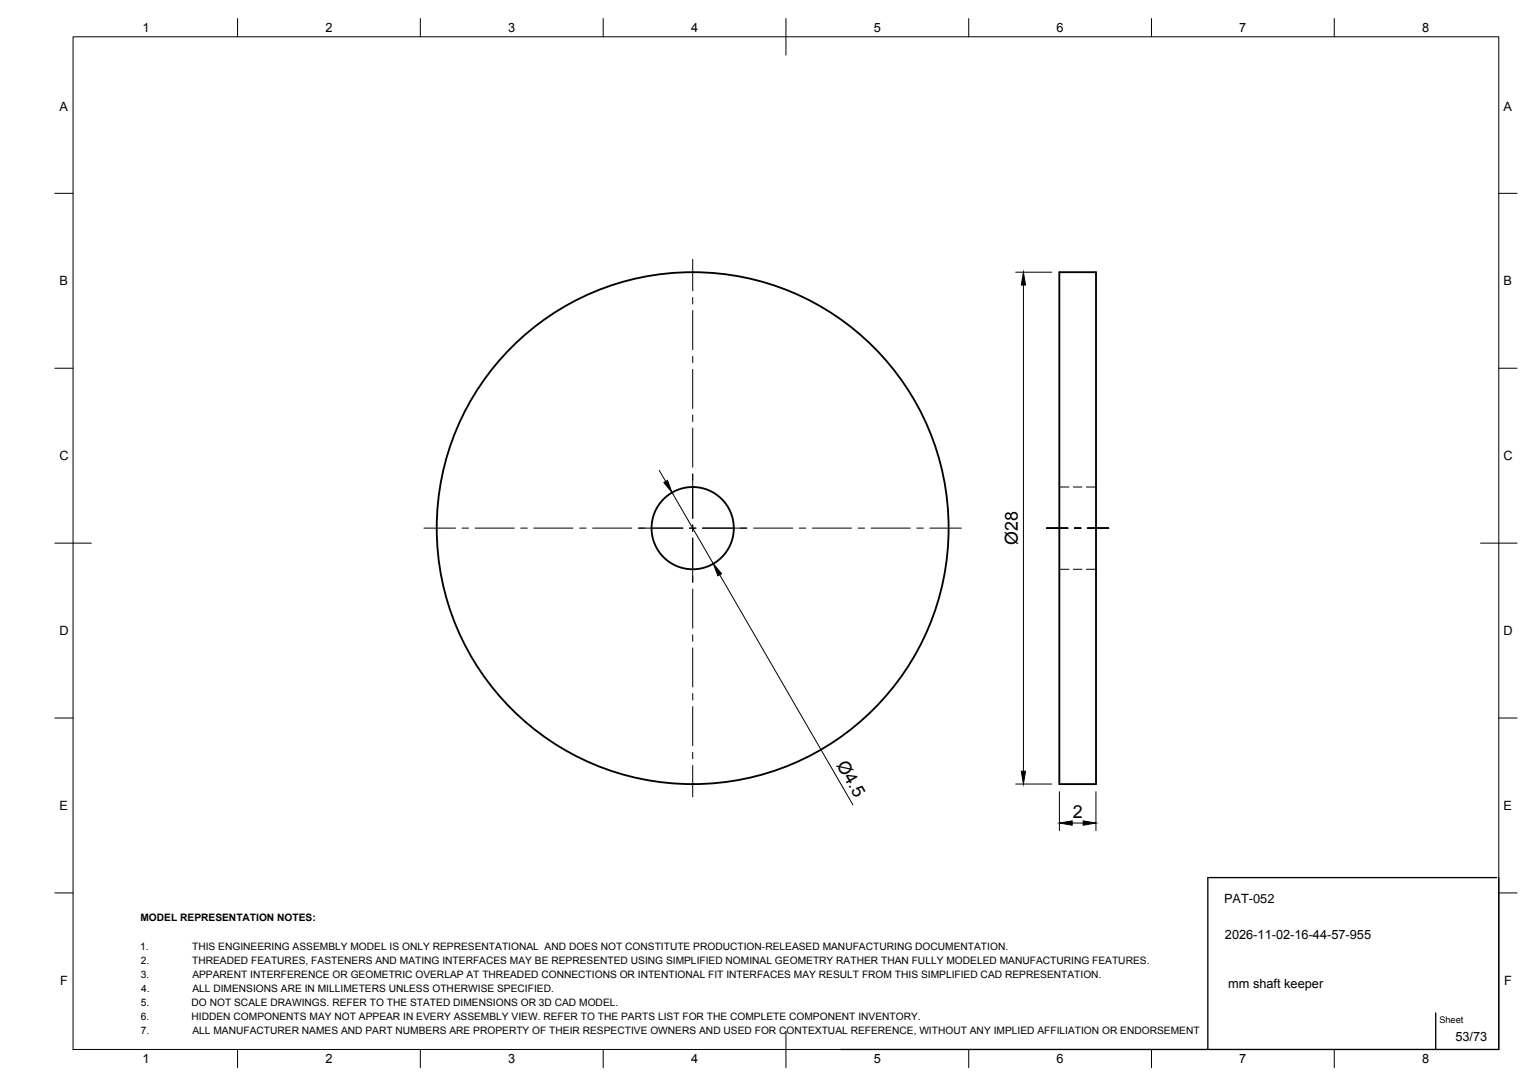
ISO-10303-21;
HEADER;
/* Generated by software containing ST-Developer
 * from STEP Tools, Inc. (www.steptools.com) 
 */

FILE_DESCRIPTION(
/* description */ ('Hand-crank gear train demonstrator'),
/* implementation_level */ '2;1');

FILE_NAME(
/* name */ 'mm shaft keeper.step',
/* time_stamp */ '2026-10-28T03:22:13-07:00',
/* author */ (''),
/* organization */ (''),
/* preprocessor_version */ 'ST-DEVELOPER v20.2',
/* originating_system */ 'Autodesk Translation Framework v15.17.0.0',
/* authorisation */ '');

FILE_SCHEMA (('AUTOMOTIVE_DESIGN { 1 0 10303 214 3 1 1 }'));
ENDSEC;

DATA;
#10=MECHANICAL_DESIGN_GEOMETRIC_PRESENTATION_REPRESENTATION('',(#1247),#62758);
#1104=SHAPE_REPRESENTATION_RELATIONSHIP('SRR','None',#63080,#1168);
#1168=ADVANCED_BREP_SHAPE_REPRESENTATION('',(#1322),#62734);
#1247=STYLED_ITEM('',(#63462),#1322);
#1322=MANIFOLD_SOLID_BREP('Body1',#16431);
#1584=FACE_BOUND('',#3842,.T.);
#1585=FACE_BOUND('',#3844,.T.);
#1955=PLANE('',#18201);
#1956=PLANE('',#18202);
#2661=FACE_OUTER_BOUND('',#3839,.T.);
#2662=FACE_OUTER_BOUND('',#3840,.T.);
#2663=FACE_OUTER_BOUND('',#3841,.T.);
#2664=FACE_OUTER_BOUND('',#3843,.T.);
#3839=EDGE_LOOP('',(#13127,#13128,#13129,#13130));
#3840=EDGE_LOOP('',(#13131,#13132,#13133,#13134));
#3841=EDGE_LOOP('',(#13135));
#3842=EDGE_LOOP('',(#13136));
#3843=EDGE_LOOP('',(#13137));
#3844=EDGE_LOOP('',(#13138));
#4953=LINE('',#26579,#6085);
#4954=LINE('',#26585,#6086);
#6085=VECTOR('',#21576,0.225);
#6086=VECTOR('',#21583,1.4);
#6989=CIRCLE('',#18196,0.225);
#6990=CIRCLE('',#18197,0.225);
#6991=CIRCLE('',#18199,1.4);
#6992=CIRCLE('',#18200,1.4);
#7990=VERTEX_POINT('',#26576);
#7991=VERTEX_POINT('',#26578);
#7992=VERTEX_POINT('',#26582);
#7993=VERTEX_POINT('',#26584);
#9815=EDGE_CURVE('',#7990,#7990,#6989,.T.);
#9816=EDGE_CURVE('',#7990,#7991,#4953,.T.);
#9817=EDGE_CURVE('',#7991,#7991,#6990,.T.);
#9818=EDGE_CURVE('',#7992,#7992,#6991,.T.);
#9819=EDGE_CURVE('',#7992,#7993,#4954,.T.);
#9820=EDGE_CURVE('',#7993,#7993,#6992,.T.);
#13127=ORIENTED_EDGE('',*,*,#9815,.F.);
#13128=ORIENTED_EDGE('',*,*,#9816,.T.);
#13129=ORIENTED_EDGE('',*,*,#9817,.T.);
#13130=ORIENTED_EDGE('',*,*,#9816,.F.);
#13131=ORIENTED_EDGE('',*,*,#9818,.F.);
#13132=ORIENTED_EDGE('',*,*,#9819,.T.);
#13133=ORIENTED_EDGE('',*,*,#9820,.T.);
#13134=ORIENTED_EDGE('',*,*,#9819,.F.);
#13135=ORIENTED_EDGE('',*,*,#9818,.T.);
#13136=ORIENTED_EDGE('',*,*,#9815,.T.);
#13137=ORIENTED_EDGE('',*,*,#9820,.F.);
#13138=ORIENTED_EDGE('',*,*,#9817,.F.);
#15329=CYLINDRICAL_SURFACE('',#18195,0.225);
#15330=CYLINDRICAL_SURFACE('',#18198,1.4);
#15971=ADVANCED_FACE('',(#2661),#15329,.F.);
#15972=ADVANCED_FACE('',(#2662),#15330,.T.);
#15973=ADVANCED_FACE('',(#2663,#1584),#1955,.T.);
#15974=ADVANCED_FACE('',(#2664,#1585),#1956,.F.);
#16431=CLOSED_SHELL('',(#15971,#15972,#15973,#15974));
#18194=AXIS2_PLACEMENT_3D('',#26574,#21570,#21571);
#18195=AXIS2_PLACEMENT_3D('',#26575,#21572,#21573);
#18196=AXIS2_PLACEMENT_3D('',#26577,#21574,#21575);
#18197=AXIS2_PLACEMENT_3D('',#26580,#21577,#21578);
#18198=AXIS2_PLACEMENT_3D('',#26581,#21579,#21580);
#18199=AXIS2_PLACEMENT_3D('',#26583,#21581,#21582);
#18200=AXIS2_PLACEMENT_3D('',#26586,#21584,#21585);
#18201=AXIS2_PLACEMENT_3D('',#26587,#21586,#21587);
#18202=AXIS2_PLACEMENT_3D('',#26588,#21588,#21589);
#21570=DIRECTION('axis',(0.,0.,1.));
#21571=DIRECTION('refdir',(1.,0.,0.));
#21572=DIRECTION('center_axis',(0.,1.,0.));
#21573=DIRECTION('ref_axis',(1.,0.,0.));
#21574=DIRECTION('center_axis',(0.,-1.,0.));
#21575=DIRECTION('ref_axis',(1.,0.,0.));
#21576=DIRECTION('',(0.,-1.,0.));
#21577=DIRECTION('center_axis',(0.,-1.,0.));
#21578=DIRECTION('ref_axis',(1.,0.,0.));
#21579=DIRECTION('center_axis',(0.,1.,0.));
#21580=DIRECTION('ref_axis',(1.,0.,0.));
#21581=DIRECTION('center_axis',(0.,1.,0.));
#21582=DIRECTION('ref_axis',(1.,0.,0.));
#21583=DIRECTION('',(0.,-1.,0.));
#21584=DIRECTION('center_axis',(0.,1.,0.));
#21585=DIRECTION('ref_axis',(1.,0.,0.));
#21586=DIRECTION('center_axis',(0.,1.,0.));
#21587=DIRECTION('ref_axis',(1.,0.,0.));
#21588=DIRECTION('center_axis',(0.,1.,0.));
#21589=DIRECTION('ref_axis',(1.,0.,0.));
#26574=CARTESIAN_POINT('',(0.,0.,0.));
#26575=CARTESIAN_POINT('Origin',(6.,3.2,9.));
#26576=CARTESIAN_POINT('',(5.775,3.4,9.));
#26577=CARTESIAN_POINT('Origin',(6.,3.4,9.));
#26578=CARTESIAN_POINT('',(5.775,3.2,9.));
#26579=CARTESIAN_POINT('',(5.775,3.2,9.));
#26580=CARTESIAN_POINT('Origin',(6.,3.2,9.));
#26581=CARTESIAN_POINT('Origin',(6.,3.2,9.));
#26582=CARTESIAN_POINT('',(4.6,3.4,9.));
#26583=CARTESIAN_POINT('Origin',(6.,3.4,9.));
#26584=CARTESIAN_POINT('',(4.6,3.2,9.));
#26585=CARTESIAN_POINT('',(4.6,3.2,9.));
#26586=CARTESIAN_POINT('Origin',(6.,3.2,9.));
#26587=CARTESIAN_POINT('Origin',(6.,3.4,9.));
#26588=CARTESIAN_POINT('Origin',(6.,3.2,9.));
#62660=UNCERTAINTY_MEASURE_WITH_UNIT(LENGTH_MEASURE(0.001),#62759,
'DISTANCE_ACCURACY_VALUE',
'Maximum model space distance between geometric entities at asserted c
onnectivities');
#62684=UNCERTAINTY_MEASURE_WITH_UNIT(LENGTH_MEASURE(0.001),#62759,
'DISTANCE_ACCURACY_VALUE',
'Maximum model space distance between geometric entities at asserted c
onnectivities');
#62734=(
GEOMETRIC_REPRESENTATION_CONTEXT(3)
GLOBAL_UNCERTAINTY_ASSIGNED_CONTEXT((#62660))
GLOBAL_UNIT_ASSIGNED_CONTEXT((#62759,#62761,#62762))
REPRESENTATION_CONTEXT('','3D')
);
#62758=(
GEOMETRIC_REPRESENTATION_CONTEXT(3)
GLOBAL_UNCERTAINTY_ASSIGNED_CONTEXT((#62684))
GLOBAL_UNIT_ASSIGNED_CONTEXT((#62759,#62761,#62762))
REPRESENTATION_CONTEXT('','3D')
);
#62759=(
LENGTH_UNIT()
NAMED_UNIT(*)
SI_UNIT(.CENTI.,.METRE.)
);
#62761=(
NAMED_UNIT(*)
PLANE_ANGLE_UNIT()
SI_UNIT($,.RADIAN.)
);
#62762=(
NAMED_UNIT(*)
SI_UNIT($,.STERADIAN.)
SOLID_ANGLE_UNIT()
);
#62812=SHAPE_DEFINITION_REPRESENTATION(#62895,#63080);
#62895=PRODUCT_DEFINITION_SHAPE('',$,#63154);
#63080=SHAPE_REPRESENTATION('',(#18194),#62734);
#63104=PRODUCT_DEFINITION_CONTEXT('part definition',#63325,'design');
#63154=PRODUCT_DEFINITION('mm shaft keeper','mm shaft keeper',#63227,#63104);
#63227=PRODUCT_DEFINITION_FORMATION('',$,#63376);
#63325=APPLICATION_CONTEXT(
'Core Data for Automotive Mechanical Design Process');
#63326=PRODUCT_CONTEXT('part definition',#63325,'mechanical');
#63376=PRODUCT('mm shaft keeper','mm shaft keeper','mm shaft keeper',(#63326));
#63456=COLOUR_RGB('Grey',0.48,0.52,0.57);
#63457=FILL_AREA_STYLE_COLOUR('',#63456);
#63458=FILL_AREA_STYLE('',(#63457));
#63459=SURFACE_STYLE_FILL_AREA(#63458);
#63460=SURFACE_SIDE_STYLE('',(#63459));
#63461=SURFACE_STYLE_USAGE(.BOTH.,#63460);
#63462=PRESENTATION_STYLE_ASSIGNMENT((#63461));
ENDSEC;
END-ISO-10303-21;
